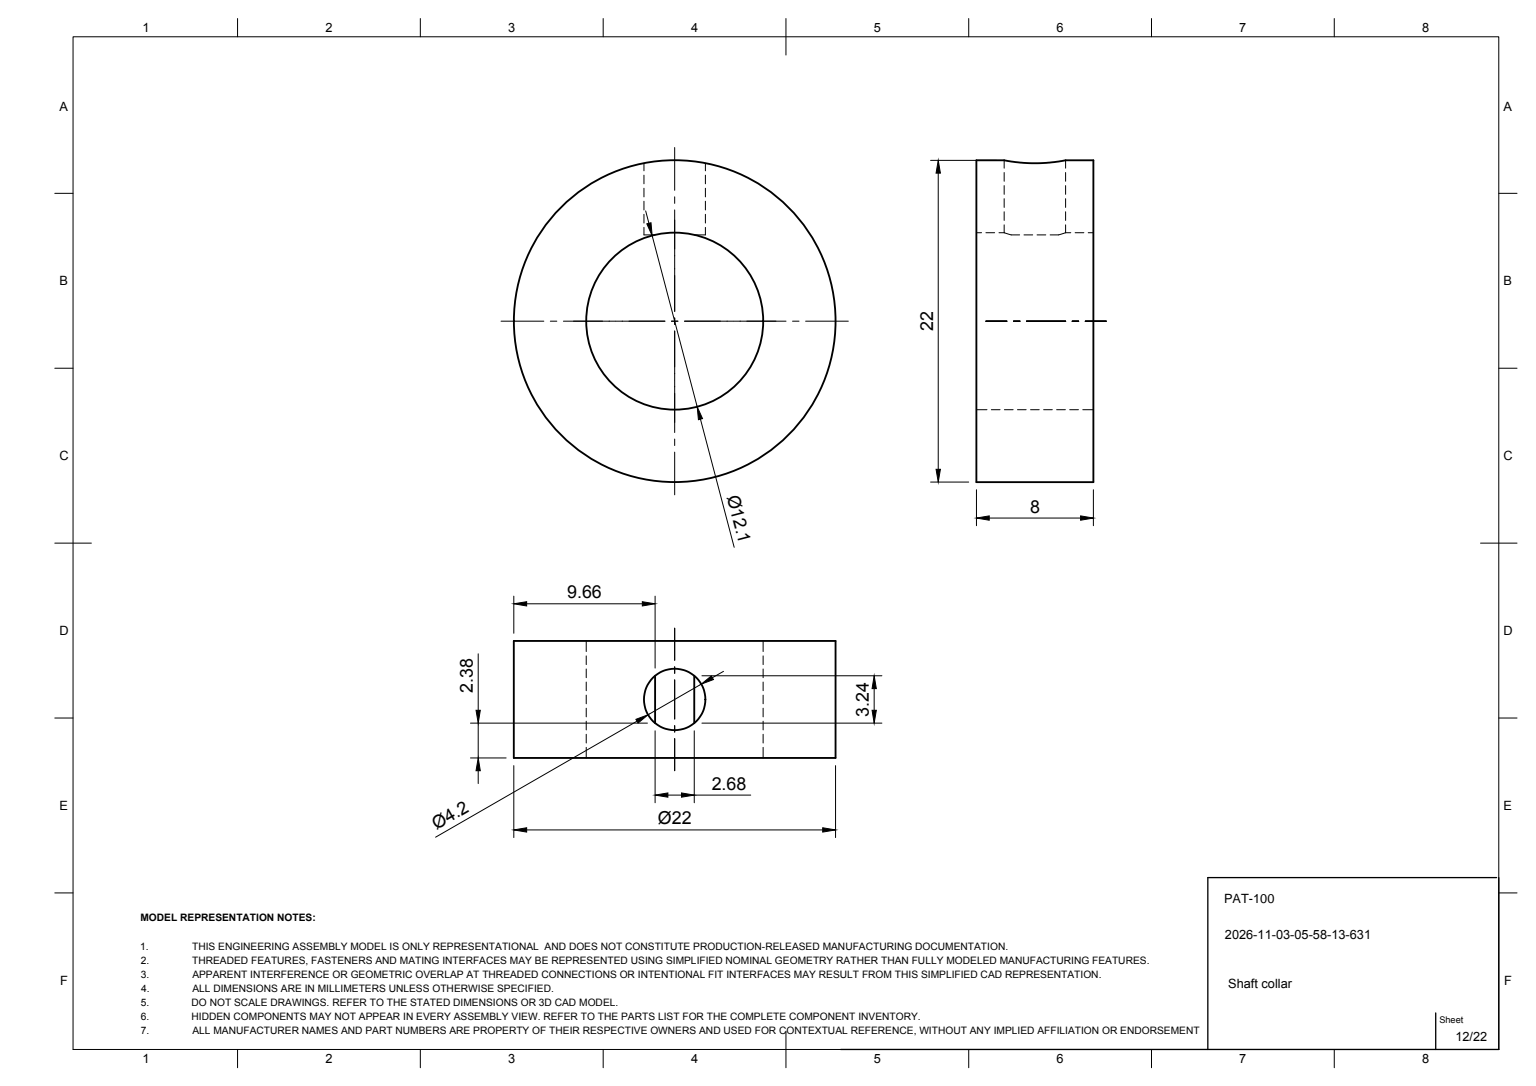
ISO-10303-21;
HEADER;
/* Generated by software containing ST-Developer
 * from STEP Tools, Inc. (www.steptools.com) 
 */

FILE_DESCRIPTION(
/* description */ (''),
/* implementation_level */ '2;1');

FILE_NAME(
/* name */ 'Shaft collar.step',
/* time_stamp */ '2026-10-29T16:43:51-07:00',
/* author */ (''),
/* organization */ (''),
/* preprocessor_version */ 'ST-DEVELOPER v20.2',
/* originating_system */ 'Autodesk Translation Framework v15.17.0.0',
/* authorisation */ '');

FILE_SCHEMA (('AUTOMOTIVE_DESIGN { 1 0 10303 214 3 1 1 }'));
ENDSEC;

DATA;
#10=MECHANICAL_DESIGN_GEOMETRIC_PRESENTATION_REPRESENTATION('',(#376),#10292);
#260=B_SPLINE_CURVE_WITH_KNOTS('',3,(#9482,#9483,#9484,#9485,#9486,#9487,
#9488,#9489,#9490,#9491),.UNSPECIFIED.,.F.,.F.,(4,2,2,2,4),(0.818088904349178,
0.878131747417165,0.957937926194036,1.03774410497091,1.09778694803889),
 .UNSPECIFIED.);
#261=B_SPLINE_CURVE_WITH_KNOTS('',3,(#9497,#9498,#9499,#9500,#9501,#9502,
#9503,#9504,#9505,#9506,#9507,#9508,#9509,#9510,#9511,#9512,#9513,#9514),
 .UNSPECIFIED.,.F.,.F.,(4,2,2,2,2,2,2,2,4),(0.,0.0793157643915218,0.158631528783044,
0.237943615933649,0.317255703084255,0.396567790234861,0.475879877385467,
0.555195641776989,0.634511406168511),.UNSPECIFIED.);
#262=B_SPLINE_CURVE_WITH_KNOTS('',3,(#9515,#9516,#9517,#9518,#9519,#9520,
#9521,#9522,#9523,#9524,#9525,#9526,#9527,#9528,#9529,#9530,#9531,#9532),
 .UNSPECIFIED.,.F.,.F.,(4,2,2,2,2,2,2,2,4),(0.634511406168511,0.713827170560032,
0.793142934951554,0.87245502210216,0.951767109252766,1.03107919640337,1.11039128355398,
1.1897070479455,1.26902281233702),.UNSPECIFIED.);
#263=B_SPLINE_CURVE_WITH_KNOTS('',3,(#9535,#9536,#9537,#9538,#9539,#9540,
#9541,#9542,#9543,#9544),.UNSPECIFIED.,.F.,.F.,(4,2,2,2,4),(0.17946362021982,
0.239506463287808,0.319312642064679,0.39911882084155,0.459161663909536),
 .UNSPECIFIED.);
#330=SHAPE_REPRESENTATION_RELATIONSHIP('SRR','None',#10426,#353);
#353=ADVANCED_BREP_SHAPE_REPRESENTATION('',(#397),#10278);
#376=STYLED_ITEM('',(#10628),#397);
#397=MANIFOLD_SOLID_BREP('Body1',#5020);
#470=FACE_BOUND('',#1208,.T.);
#471=FACE_BOUND('',#1210,.T.);
#472=FACE_BOUND('',#1212,.T.);
#473=FACE_BOUND('',#1214,.T.);
#621=PLANE('',#5536);
#622=PLANE('',#5541);
#623=PLANE('',#5548);
#624=PLANE('',#5549);
#852=FACE_OUTER_BOUND('',#1204,.T.);
#853=FACE_OUTER_BOUND('',#1205,.T.);
#854=FACE_OUTER_BOUND('',#1206,.T.);
#855=FACE_OUTER_BOUND('',#1207,.T.);
#856=FACE_OUTER_BOUND('',#1209,.T.);
#857=FACE_OUTER_BOUND('',#1211,.T.);
#858=FACE_OUTER_BOUND('',#1213,.T.);
#1204=EDGE_LOOP('',(#4045,#4046));
#1205=EDGE_LOOP('',(#4047,#4048,#4049,#4050,#4051,#4052,#4053,#4054,#4055));
#1206=EDGE_LOOP('',(#4056,#4057,#4058));
#1207=EDGE_LOOP('',(#4059,#4060,#4061,#4062));
#1208=EDGE_LOOP('',(#4063,#4064,#4065,#4066));
#1209=EDGE_LOOP('',(#4067,#4068,#4069,#4070));
#1210=EDGE_LOOP('',(#4071,#4072));
#1211=EDGE_LOOP('',(#4073));
#1212=EDGE_LOOP('',(#4074));
#1213=EDGE_LOOP('',(#4075));
#1214=EDGE_LOOP('',(#4076));
#1618=LINE('',#9478,#2010);
#1619=LINE('',#9495,#2011);
#1620=LINE('',#9546,#2012);
#1621=LINE('',#9551,#2013);
#1622=LINE('',#9557,#2014);
#2010=VECTOR('',#6567,1.);
#2011=VECTOR('',#6574,0.21);
#2012=VECTOR('',#6579,1.);
#2013=VECTOR('',#6584,0.605);
#2014=VECTOR('',#6591,1.1);
#2287=CIRCLE('',#5537,0.21);
#2288=CIRCLE('',#5539,0.21);
#2289=CIRCLE('',#5540,0.21);
#2290=CIRCLE('',#5543,0.605);
#2291=CIRCLE('',#5544,0.605);
#2292=CIRCLE('',#5546,1.1);
#2293=CIRCLE('',#5547,1.1);
#2602=VERTEX_POINT('',#9476);
#2603=VERTEX_POINT('',#9477);
#2604=VERTEX_POINT('',#9481);
#2605=VERTEX_POINT('',#9492);
#2606=VERTEX_POINT('',#9494);
#2607=VERTEX_POINT('',#9496);
#2608=VERTEX_POINT('',#9533);
#2609=VERTEX_POINT('',#9548);
#2610=VERTEX_POINT('',#9550);
#2611=VERTEX_POINT('',#9554);
#2612=VERTEX_POINT('',#9556);
#3113=EDGE_CURVE('',#2602,#2603,#1618,.T.);
#3114=EDGE_CURVE('',#2602,#2603,#2287,.T.);
#3115=EDGE_CURVE('',#2604,#2602,#260,.T.);
#3116=EDGE_CURVE('',#2605,#2604,#2288,.T.);
#3117=EDGE_CURVE('',#2605,#2606,#1619,.T.);
#3118=EDGE_CURVE('',#2607,#2606,#261,.T.);
#3119=EDGE_CURVE('',#2606,#2607,#262,.T.);
#3120=EDGE_CURVE('',#2608,#2605,#2289,.T.);
#3121=EDGE_CURVE('',#2603,#2608,#263,.T.);
#3122=EDGE_CURVE('',#2608,#2604,#1620,.T.);
#3123=EDGE_CURVE('',#2609,#2609,#2290,.T.);
#3124=EDGE_CURVE('',#2609,#2610,#1621,.T.);
#3125=EDGE_CURVE('',#2610,#2610,#2291,.T.);
#3126=EDGE_CURVE('',#2611,#2611,#2292,.T.);
#3127=EDGE_CURVE('',#2611,#2612,#1622,.T.);
#3128=EDGE_CURVE('',#2612,#2612,#2293,.T.);
#4045=ORIENTED_EDGE('',*,*,#3113,.F.);
#4046=ORIENTED_EDGE('',*,*,#3114,.T.);
#4047=ORIENTED_EDGE('',*,*,#3115,.F.);
#4048=ORIENTED_EDGE('',*,*,#3116,.F.);
#4049=ORIENTED_EDGE('',*,*,#3117,.T.);
#4050=ORIENTED_EDGE('',*,*,#3118,.F.);
#4051=ORIENTED_EDGE('',*,*,#3119,.F.);
#4052=ORIENTED_EDGE('',*,*,#3117,.F.);
#4053=ORIENTED_EDGE('',*,*,#3120,.F.);
#4054=ORIENTED_EDGE('',*,*,#3121,.F.);
#4055=ORIENTED_EDGE('',*,*,#3114,.F.);
#4056=ORIENTED_EDGE('',*,*,#3122,.F.);
#4057=ORIENTED_EDGE('',*,*,#3120,.T.);
#4058=ORIENTED_EDGE('',*,*,#3116,.T.);
#4059=ORIENTED_EDGE('',*,*,#3123,.F.);
#4060=ORIENTED_EDGE('',*,*,#3124,.T.);
#4061=ORIENTED_EDGE('',*,*,#3125,.T.);
#4062=ORIENTED_EDGE('',*,*,#3124,.F.);
#4063=ORIENTED_EDGE('',*,*,#3121,.T.);
#4064=ORIENTED_EDGE('',*,*,#3122,.T.);
#4065=ORIENTED_EDGE('',*,*,#3115,.T.);
#4066=ORIENTED_EDGE('',*,*,#3113,.T.);
#4067=ORIENTED_EDGE('',*,*,#3126,.F.);
#4068=ORIENTED_EDGE('',*,*,#3127,.T.);
#4069=ORIENTED_EDGE('',*,*,#3128,.T.);
#4070=ORIENTED_EDGE('',*,*,#3127,.F.);
#4071=ORIENTED_EDGE('',*,*,#3118,.T.);
#4072=ORIENTED_EDGE('',*,*,#3119,.T.);
#4073=ORIENTED_EDGE('',*,*,#3126,.T.);
#4074=ORIENTED_EDGE('',*,*,#3123,.T.);
#4075=ORIENTED_EDGE('',*,*,#3128,.F.);
#4076=ORIENTED_EDGE('',*,*,#3125,.F.);
#4676=CYLINDRICAL_SURFACE('',#5538,0.21);
#4677=CYLINDRICAL_SURFACE('',#5542,0.605);
#4678=CYLINDRICAL_SURFACE('',#5545,1.1);
#4861=ADVANCED_FACE('',(#852),#621,.T.);
#4862=ADVANCED_FACE('',(#853),#4676,.F.);
#4863=ADVANCED_FACE('',(#854),#622,.T.);
#4864=ADVANCED_FACE('',(#855,#470),#4677,.F.);
#4865=ADVANCED_FACE('',(#856,#471),#4678,.T.);
#4866=ADVANCED_FACE('',(#857,#472),#623,.T.);
#4867=ADVANCED_FACE('',(#858,#473),#624,.F.);
#5020=CLOSED_SHELL('',(#4861,#4862,#4863,#4864,#4865,#4866,#4867));
#5535=AXIS2_PLACEMENT_3D('',#9474,#6563,#6564);
#5536=AXIS2_PLACEMENT_3D('',#9475,#6565,#6566);
#5537=AXIS2_PLACEMENT_3D('',#9479,#6568,#6569);
#5538=AXIS2_PLACEMENT_3D('',#9480,#6570,#6571);
#5539=AXIS2_PLACEMENT_3D('',#9493,#6572,#6573);
#5540=AXIS2_PLACEMENT_3D('',#9534,#6575,#6576);
#5541=AXIS2_PLACEMENT_3D('',#9545,#6577,#6578);
#5542=AXIS2_PLACEMENT_3D('',#9547,#6580,#6581);
#5543=AXIS2_PLACEMENT_3D('',#9549,#6582,#6583);
#5544=AXIS2_PLACEMENT_3D('',#9552,#6585,#6586);
#5545=AXIS2_PLACEMENT_3D('',#9553,#6587,#6588);
#5546=AXIS2_PLACEMENT_3D('',#9555,#6589,#6590);
#5547=AXIS2_PLACEMENT_3D('',#9558,#6592,#6593);
#5548=AXIS2_PLACEMENT_3D('',#9559,#6594,#6595);
#5549=AXIS2_PLACEMENT_3D('',#9560,#6596,#6597);
#6563=DIRECTION('axis',(0.,0.,1.));
#6564=DIRECTION('refdir',(1.,0.,0.));
#6565=DIRECTION('center_axis',(0.,0.,1.));
#6566=DIRECTION('ref_axis',(1.,0.,0.));
#6567=DIRECTION('',(0.,1.,0.));
#6568=DIRECTION('center_axis',(0.,0.,1.));
#6569=DIRECTION('ref_axis',(1.,0.,0.));
#6570=DIRECTION('center_axis',(0.,0.,1.));
#6571=DIRECTION('ref_axis',(1.,0.,0.));
#6572=DIRECTION('center_axis',(0.,0.,1.));
#6573=DIRECTION('ref_axis',(1.,0.,0.));
#6574=DIRECTION('',(0.,0.,1.));
#6575=DIRECTION('center_axis',(0.,0.,1.));
#6576=DIRECTION('ref_axis',(1.,0.,0.));
#6577=DIRECTION('center_axis',(0.,0.,1.));
#6578=DIRECTION('ref_axis',(1.,0.,0.));
#6579=DIRECTION('',(0.,-1.,0.));
#6580=DIRECTION('center_axis',(0.,1.,0.));
#6581=DIRECTION('ref_axis',(1.,0.,0.));
#6582=DIRECTION('center_axis',(0.,-1.,0.));
#6583=DIRECTION('ref_axis',(1.,0.,0.));
#6584=DIRECTION('',(0.,-1.,0.));
#6585=DIRECTION('center_axis',(0.,-1.,0.));
#6586=DIRECTION('ref_axis',(1.,0.,0.));
#6587=DIRECTION('center_axis',(0.,1.,0.));
#6588=DIRECTION('ref_axis',(1.,0.,0.));
#6589=DIRECTION('center_axis',(0.,1.,0.));
#6590=DIRECTION('ref_axis',(1.,0.,0.));
#6591=DIRECTION('',(0.,-1.,0.));
#6592=DIRECTION('center_axis',(0.,1.,0.));
#6593=DIRECTION('ref_axis',(1.,0.,0.));
#6594=DIRECTION('center_axis',(0.,1.,0.));
#6595=DIRECTION('ref_axis',(1.,0.,0.));
#6596=DIRECTION('center_axis',(0.,1.,0.));
#6597=DIRECTION('ref_axis',(1.,0.,0.));
#9474=CARTESIAN_POINT('',(0.,0.,0.));
#9475=CARTESIAN_POINT('Origin',(0.,5.3,10.59));
#9476=CARTESIAN_POINT('',(0.133884278389952,5.13821310312636,10.59));
#9477=CARTESIAN_POINT('',(0.133884278389952,5.46178689687364,10.59));
#9478=CARTESIAN_POINT('',(0.133884278389952,4.9,10.59));
#9479=CARTESIAN_POINT('Origin',(0.,5.3,10.59));
#9480=CARTESIAN_POINT('Origin',(0.,5.3,10.59));
#9481=CARTESIAN_POINT('',(-0.133884278389952,5.13821310312636,10.59));
#9482=CARTESIAN_POINT('Ctrl Pts',(-0.133884278389952,5.13821310312636,10.59));
#9483=CARTESIAN_POINT('Ctrl Pts',(-0.118254395260799,5.12527883178237,10.5935467722442));
#9484=CARTESIAN_POINT('Ctrl Pts',(-0.100109787682297,5.11420068341256,10.5969822478996));
#9485=CARTESIAN_POINT('Ctrl Pts',(-0.0548298721325188,5.09536143894557,
10.6030741628997));
#9486=CARTESIAN_POINT('Ctrl Pts',(-0.0266020595922903,5.09,10.605));
#9487=CARTESIAN_POINT('Ctrl Pts',(0.0266020595922903,5.09,10.605));
#9488=CARTESIAN_POINT('Ctrl Pts',(0.0548298721325188,5.09536143894557,10.6030741628997));
#9489=CARTESIAN_POINT('Ctrl Pts',(0.100109787682297,5.11420068341256,10.5969822478996));
#9490=CARTESIAN_POINT('Ctrl Pts',(0.118254395260799,5.12527883178237,10.5935467722442));
#9491=CARTESIAN_POINT('Ctrl Pts',(0.133884278389952,5.13821310312636,10.59));
#9492=CARTESIAN_POINT('',(-0.21,5.3,10.59));
#9493=CARTESIAN_POINT('Origin',(0.,5.3,10.59));
#9494=CARTESIAN_POINT('',(-0.21,5.3,11.0797684937059));
#9495=CARTESIAN_POINT('',(-0.21,5.3,10.59));
#9496=CARTESIAN_POINT('',(0.21,5.3,11.0797684937059));
#9497=CARTESIAN_POINT('Ctrl Pts',(0.21,5.3,11.0797684937059));
#9498=CARTESIAN_POINT('Ctrl Pts',(0.21,5.27356141186949,11.0797684937059));
#9499=CARTESIAN_POINT('Ctrl Pts',(0.204702922670976,5.24540621874507,11.0808401566467));
#9500=CARTESIAN_POINT('Ctrl Pts',(0.183251796806354,5.19368655445866,11.0846831370713));
#9501=CARTESIAN_POINT('Ctrl Pts',(0.167101177357215,5.17011632925886,11.0873959305462));
#9502=CARTESIAN_POINT('Ctrl Pts',(0.129884533480965,5.13289968538261,11.0924663328912));
#9503=CARTESIAN_POINT('Ctrl Pts',(0.106313940757289,5.11674838983659,11.0951573889536));
#9504=CARTESIAN_POINT('Ctrl Pts',(0.0545930033295207,5.09529677343026,11.0989503922059));
#9505=CARTESIAN_POINT('Ctrl Pts',(0.0264373623835353,5.09,11.1));
#9506=CARTESIAN_POINT('Ctrl Pts',(-0.0264373623835352,5.09,11.1));
#9507=CARTESIAN_POINT('Ctrl Pts',(-0.0545930033295207,5.09529677343026,
11.0989503922059));
#9508=CARTESIAN_POINT('Ctrl Pts',(-0.106313940757289,5.11674838983659,11.0951573889536));
#9509=CARTESIAN_POINT('Ctrl Pts',(-0.129884533480965,5.13289968538261,11.0924663328912));
#9510=CARTESIAN_POINT('Ctrl Pts',(-0.167101177357215,5.17011632925886,11.0873959305462));
#9511=CARTESIAN_POINT('Ctrl Pts',(-0.183251796806354,5.19368655445866,11.0846831370713));
#9512=CARTESIAN_POINT('Ctrl Pts',(-0.204702922670976,5.24540621874507,11.0808401566467));
#9513=CARTESIAN_POINT('Ctrl Pts',(-0.21,5.27356141186949,11.0797684937059));
#9514=CARTESIAN_POINT('Ctrl Pts',(-0.21,5.3,11.0797684937059));
#9515=CARTESIAN_POINT('Ctrl Pts',(-0.21,5.3,11.0797684937059));
#9516=CARTESIAN_POINT('Ctrl Pts',(-0.21,5.32643858813051,11.0797684937059));
#9517=CARTESIAN_POINT('Ctrl Pts',(-0.204702922670976,5.35459378125493,11.0808401566467));
#9518=CARTESIAN_POINT('Ctrl Pts',(-0.183251796806354,5.40631344554134,11.0846831370713));
#9519=CARTESIAN_POINT('Ctrl Pts',(-0.167101177357215,5.42988367074114,11.0873959305462));
#9520=CARTESIAN_POINT('Ctrl Pts',(-0.129884533480965,5.46710031461738,11.0924663328912));
#9521=CARTESIAN_POINT('Ctrl Pts',(-0.106313940757289,5.48325161016341,11.0951573889536));
#9522=CARTESIAN_POINT('Ctrl Pts',(-0.0545930033295208,5.50470322656974,
11.0989503922059));
#9523=CARTESIAN_POINT('Ctrl Pts',(-0.0264373623835353,5.51,11.1));
#9524=CARTESIAN_POINT('Ctrl Pts',(0.0264373623835352,5.51,11.1));
#9525=CARTESIAN_POINT('Ctrl Pts',(0.0545930033295208,5.50470322656974,11.0989503922059));
#9526=CARTESIAN_POINT('Ctrl Pts',(0.106313940757289,5.48325161016341,11.0951573889536));
#9527=CARTESIAN_POINT('Ctrl Pts',(0.129884533480965,5.46710031461738,11.0924663328912));
#9528=CARTESIAN_POINT('Ctrl Pts',(0.167101177357214,5.42988367074114,11.0873959305462));
#9529=CARTESIAN_POINT('Ctrl Pts',(0.183251796806354,5.40631344554134,11.0846831370713));
#9530=CARTESIAN_POINT('Ctrl Pts',(0.204702922670976,5.35459378125493,11.0808401566467));
#9531=CARTESIAN_POINT('Ctrl Pts',(0.21,5.32643858813051,11.0797684937059));
#9532=CARTESIAN_POINT('Ctrl Pts',(0.21,5.3,11.0797684937059));
#9533=CARTESIAN_POINT('',(-0.133884278389952,5.46178689687364,10.59));
#9534=CARTESIAN_POINT('Origin',(0.,5.3,10.59));
#9535=CARTESIAN_POINT('Ctrl Pts',(0.133884278389952,5.46178689687364,10.59));
#9536=CARTESIAN_POINT('Ctrl Pts',(0.118254395260798,5.47472116821763,10.5935467722442));
#9537=CARTESIAN_POINT('Ctrl Pts',(0.100109787682297,5.48579931658744,10.5969822478996));
#9538=CARTESIAN_POINT('Ctrl Pts',(0.0548298721325188,5.50463856105443,10.6030741628997));
#9539=CARTESIAN_POINT('Ctrl Pts',(0.0266020595922903,5.51,10.605));
#9540=CARTESIAN_POINT('Ctrl Pts',(-0.0266020595922903,5.51,10.605));
#9541=CARTESIAN_POINT('Ctrl Pts',(-0.0548298721325188,5.50463856105443,
10.6030741628997));
#9542=CARTESIAN_POINT('Ctrl Pts',(-0.100109787682297,5.48579931658744,10.5969822478996));
#9543=CARTESIAN_POINT('Ctrl Pts',(-0.118254395260799,5.47472116821763,10.5935467722442));
#9544=CARTESIAN_POINT('Ctrl Pts',(-0.133884278389952,5.46178689687364,10.59));
#9545=CARTESIAN_POINT('Origin',(0.,5.3,10.59));
#9546=CARTESIAN_POINT('',(-0.133884278389952,4.9,10.59));
#9547=CARTESIAN_POINT('Origin',(0.,4.9,10.));
#9548=CARTESIAN_POINT('',(-0.605,5.7,10.));
#9549=CARTESIAN_POINT('Origin',(0.,5.7,10.));
#9550=CARTESIAN_POINT('',(-0.605,4.9,10.));
#9551=CARTESIAN_POINT('',(-0.605,4.9,10.));
#9552=CARTESIAN_POINT('Origin',(0.,4.9,10.));
#9553=CARTESIAN_POINT('Origin',(0.,4.9,10.));
#9554=CARTESIAN_POINT('',(-1.1,5.7,10.));
#9555=CARTESIAN_POINT('Origin',(0.,5.7,10.));
#9556=CARTESIAN_POINT('',(-1.1,4.9,10.));
#9557=CARTESIAN_POINT('',(-1.1,4.9,10.));
#9558=CARTESIAN_POINT('Origin',(0.,4.9,10.));
#9559=CARTESIAN_POINT('Origin',(0.,5.7,10.));
#9560=CARTESIAN_POINT('Origin',(0.,4.9,10.));
#10250=UNCERTAINTY_MEASURE_WITH_UNIT(LENGTH_MEASURE(0.001),#10293,
'DISTANCE_ACCURACY_VALUE',
'Maximum model space distance between geometric entities at asserted c
onnectivities');
#10264=UNCERTAINTY_MEASURE_WITH_UNIT(LENGTH_MEASURE(0.001),#10293,
'DISTANCE_ACCURACY_VALUE',
'Maximum model space distance between geometric entities at asserted c
onnectivities');
#10278=(
GEOMETRIC_REPRESENTATION_CONTEXT(3)
GLOBAL_UNCERTAINTY_ASSIGNED_CONTEXT((#10250))
GLOBAL_UNIT_ASSIGNED_CONTEXT((#10293,#10295,#10296))
REPRESENTATION_CONTEXT('','3D')
);
#10292=(
GEOMETRIC_REPRESENTATION_CONTEXT(3)
GLOBAL_UNCERTAINTY_ASSIGNED_CONTEXT((#10264))
GLOBAL_UNIT_ASSIGNED_CONTEXT((#10293,#10295,#10296))
REPRESENTATION_CONTEXT('','3D')
);
#10293=(
LENGTH_UNIT()
NAMED_UNIT(*)
SI_UNIT(.CENTI.,.METRE.)
);
#10295=(
NAMED_UNIT(*)
PLANE_ANGLE_UNIT()
SI_UNIT($,.RADIAN.)
);
#10296=(
NAMED_UNIT(*)
SI_UNIT($,.STERADIAN.)
SOLID_ANGLE_UNIT()
);
#10310=SHAPE_DEFINITION_REPRESENTATION(#10337,#10426);
#10337=PRODUCT_DEFINITION_SHAPE('',$,#10454);
#10426=SHAPE_REPRESENTATION('',(#5535),#10278);
#10440=PRODUCT_DEFINITION_CONTEXT('part definition',#10523,'design');
#10454=PRODUCT_DEFINITION('Shaft collar','Shaft collar',#10481,
#10440);
#10481=PRODUCT_DEFINITION_FORMATION('',$,#10538);
#10523=APPLICATION_CONTEXT(
'Core Data for Automotive Mechanical Design Process');
#10524=PRODUCT_CONTEXT('part definition',#10523,'mechanical');
#10538=PRODUCT('Shaft collar','Shaft collar','Shaft collar',
(#10524));
#10622=COLOUR_RGB('Grey',0.48,0.52,0.57);
#10623=FILL_AREA_STYLE_COLOUR('',#10622);
#10624=FILL_AREA_STYLE('',(#10623));
#10625=SURFACE_STYLE_FILL_AREA(#10624);
#10626=SURFACE_SIDE_STYLE('',(#10625));
#10627=SURFACE_STYLE_USAGE(.BOTH.,#10626);
#10628=PRESENTATION_STYLE_ASSIGNMENT((#10627));
ENDSEC;
END-ISO-10303-21;
